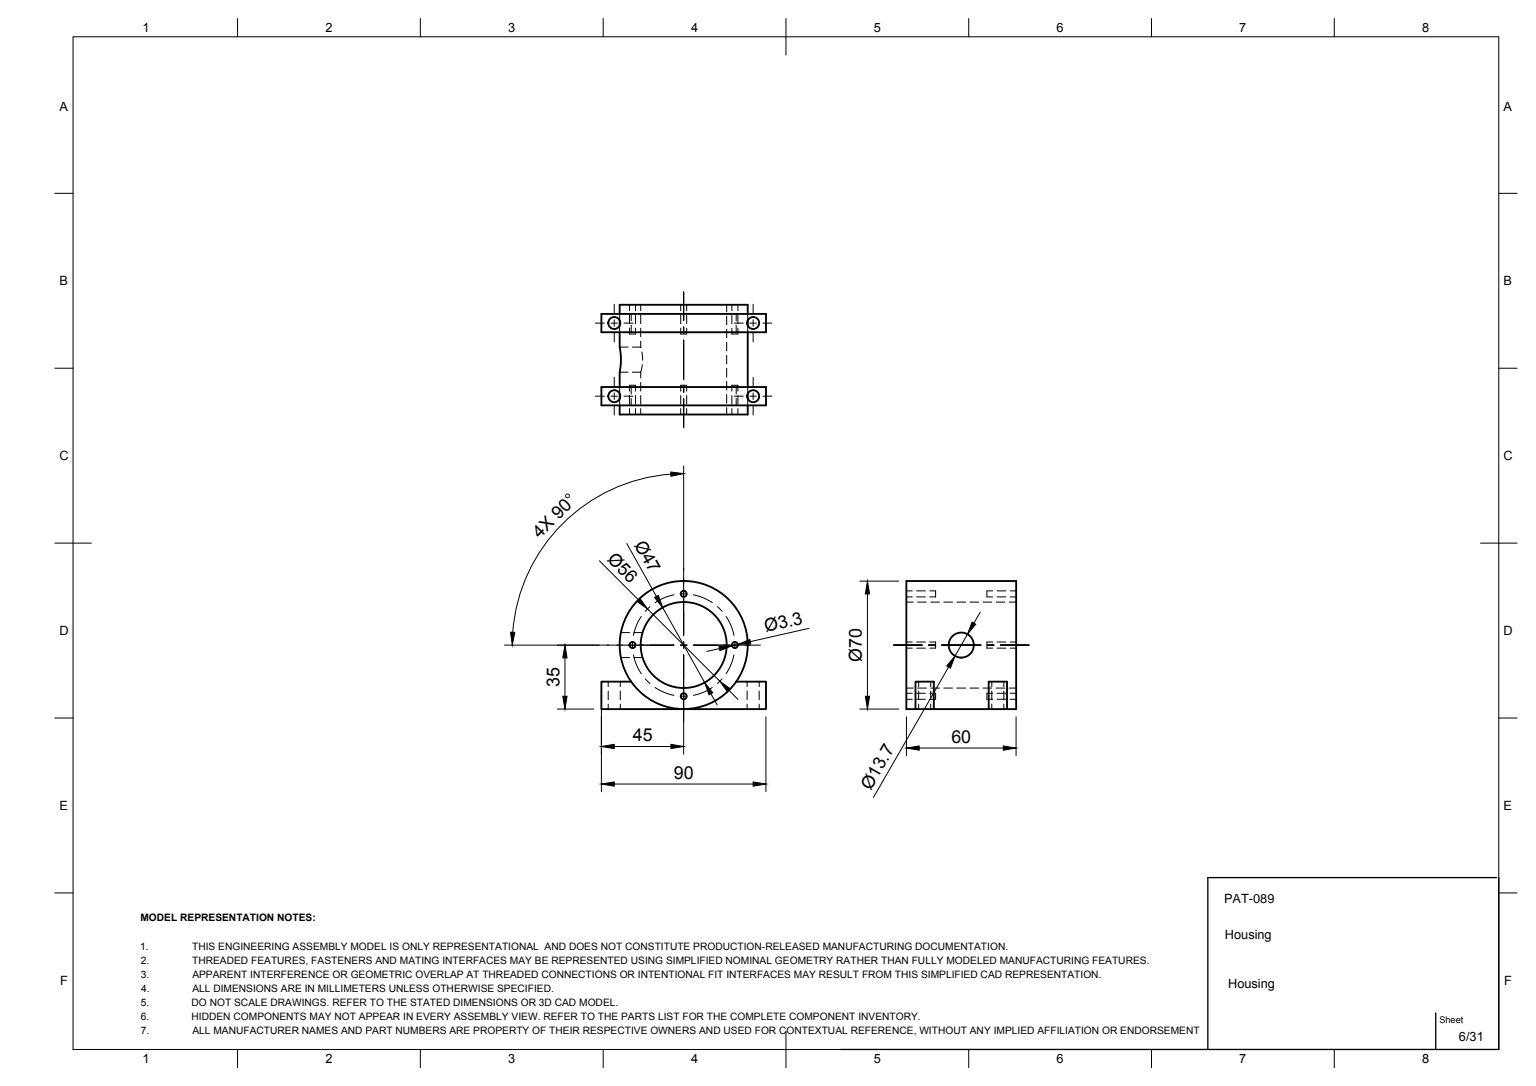
ISO-10303-21;
HEADER;
/* Generated by software containing ST-Developer
 * from STEP Tools, Inc. (www.steptools.com) 
 */

FILE_DESCRIPTION(
/* description */ ('Rotary union on bearing shaft'),
/* implementation_level */ '2;1');

FILE_NAME(
/* name */ 'Housing.step',
/* time_stamp */ '2026-10-28T03:24:01-07:00',
/* author */ (''),
/* organization */ (''),
/* preprocessor_version */ 'ST-DEVELOPER v20.2',
/* originating_system */ 'Autodesk Translation Framework v15.17.0.0',
/* authorisation */ '');

FILE_SCHEMA (('AUTOMOTIVE_DESIGN { 1 0 10303 214 3 1 1 }'));
ENDSEC;

DATA;
#10=MECHANICAL_DESIGN_GEOMETRIC_PRESENTATION_REPRESENTATION('',(#314),#9448);
#225=B_SPLINE_CURVE_WITH_KNOTS('',3,(#7509,#7510,#7511,#7512,#7513,#7514,
#7515,#7516,#7517,#7518,#7519,#7520,#7521,#7522,#7523,#7524,#7525,#7526),
 .UNSPECIFIED.,.F.,.F.,(4,2,2,2,2,2,2,2,4),(0.,0.259699157802782,0.519398315605563,
0.779028864963069,1.03865941432058,1.29828996367808,1.55792051303559,1.81761967083837,
2.07731882864115),.UNSPECIFIED.);
#226=B_SPLINE_CURVE_WITH_KNOTS('',3,(#7527,#7528,#7529,#7530,#7531,#7532,
#7533,#7534,#7535,#7536,#7537,#7538,#7539,#7540,#7541,#7542,#7543,#7544),
 .UNSPECIFIED.,.F.,.F.,(4,2,2,2,2,2,2,2,4),(2.07731882864115,2.33701798644393,
2.59671714424671,2.85634769360422,3.11597824296173,3.37560879231923,3.63523934167674,
3.89493849947952,4.1546376572823),.UNSPECIFIED.);
#227=B_SPLINE_CURVE_WITH_KNOTS('',3,(#7548,#7549,#7550,#7551,#7552,#7553,
#7554,#7555,#7556,#7557,#7558,#7559,#7560,#7561,#7562,#7563,#7564,#7565),
 .UNSPECIFIED.,.F.,.F.,(4,2,2,2,2,2,2,2,4),(0.,0.258756642336745,0.51751328467349,
0.776256652721243,1.035000020769,1.29374338881675,1.5524867568645,1.81124339920125,
2.07000004153799),.UNSPECIFIED.);
#228=B_SPLINE_CURVE_WITH_KNOTS('',3,(#7566,#7567,#7568,#7569,#7570,#7571,
#7572,#7573,#7574,#7575,#7576,#7577,#7578,#7579,#7580,#7581,#7582,#7583),
 .UNSPECIFIED.,.F.,.F.,(4,2,2,2,2,2,2,2,4),(2.07000004153799,2.32875668387474,
2.58751332621148,2.84625669425923,3.10500006230699,3.36374343035474,3.62248679840249,
3.88124344073924,4.14000008307598),.UNSPECIFIED.);
#260=SHAPE_REPRESENTATION_RELATIONSHIP('SRR','None',#9560,#287);
#287=ADVANCED_BREP_SHAPE_REPRESENTATION('',(#349),#9420);
#314=STYLED_ITEM('',(#9757),#349);
#349=MANIFOLD_SOLID_BREP('Body1',#4869);
#388=FACE_BOUND('',#999,.T.);
#389=FACE_BOUND('',#1001,.T.);
#390=FACE_BOUND('',#1004,.T.);
#391=FACE_BOUND('',#1005,.T.);
#392=FACE_BOUND('',#1012,.T.);
#393=FACE_BOUND('',#1014,.T.);
#394=FACE_BOUND('',#1017,.T.);
#395=FACE_BOUND('',#1018,.T.);
#396=FACE_BOUND('',#1021,.T.);
#397=FACE_BOUND('',#1023,.T.);
#398=FACE_BOUND('',#1024,.T.);
#399=FACE_BOUND('',#1025,.T.);
#400=FACE_BOUND('',#1027,.T.);
#401=FACE_BOUND('',#1028,.T.);
#402=FACE_BOUND('',#1029,.T.);
#403=FACE_BOUND('',#1030,.T.);
#404=FACE_BOUND('',#1031,.T.);
#405=FACE_BOUND('',#1033,.T.);
#406=FACE_BOUND('',#1034,.T.);
#407=FACE_BOUND('',#1035,.T.);
#408=FACE_BOUND('',#1036,.T.);
#409=FACE_BOUND('',#1037,.T.);
#493=PLANE('',#5229);
#494=PLANE('',#5233);
#495=PLANE('',#5237);
#496=PLANE('',#5241);
#497=PLANE('',#5245);
#498=PLANE('',#5249);
#499=PLANE('',#5253);
#500=PLANE('',#5257);
#501=PLANE('',#5271);
#502=PLANE('',#5273);
#503=PLANE('',#5275);
#504=PLANE('',#5277);
#505=PLANE('',#5279);
#506=PLANE('',#5280);
#507=PLANE('',#5281);
#508=PLANE('',#5282);
#509=PLANE('',#5283);
#510=PLANE('',#5284);
#511=PLANE('',#5286);
#512=PLANE('',#5288);
#513=PLANE('',#5290);
#514=PLANE('',#5292);
#515=PLANE('',#5293);
#516=PLANE('',#5294);
#517=PLANE('',#5295);
#518=PLANE('',#5296);
#519=PLANE('',#5303);
#520=PLANE('',#5304);
#666=FACE_OUTER_BOUND('',#973,.T.);
#667=FACE_OUTER_BOUND('',#974,.T.);
#668=FACE_OUTER_BOUND('',#975,.T.);
#669=FACE_OUTER_BOUND('',#976,.T.);
#670=FACE_OUTER_BOUND('',#977,.T.);
#671=FACE_OUTER_BOUND('',#978,.T.);
#672=FACE_OUTER_BOUND('',#979,.T.);
#673=FACE_OUTER_BOUND('',#980,.T.);
#674=FACE_OUTER_BOUND('',#981,.T.);
#675=FACE_OUTER_BOUND('',#982,.T.);
#676=FACE_OUTER_BOUND('',#983,.T.);
#677=FACE_OUTER_BOUND('',#984,.T.);
#678=FACE_OUTER_BOUND('',#985,.T.);
#679=FACE_OUTER_BOUND('',#986,.T.);
#680=FACE_OUTER_BOUND('',#987,.T.);
#681=FACE_OUTER_BOUND('',#988,.T.);
#682=FACE_OUTER_BOUND('',#989,.T.);
#683=FACE_OUTER_BOUND('',#990,.T.);
#684=FACE_OUTER_BOUND('',#991,.T.);
#685=FACE_OUTER_BOUND('',#992,.T.);
#686=FACE_OUTER_BOUND('',#993,.T.);
#687=FACE_OUTER_BOUND('',#994,.T.);
#688=FACE_OUTER_BOUND('',#995,.T.);
#689=FACE_OUTER_BOUND('',#996,.T.);
#690=FACE_OUTER_BOUND('',#997,.T.);
#691=FACE_OUTER_BOUND('',#998,.T.);
#692=FACE_OUTER_BOUND('',#1000,.T.);
#693=FACE_OUTER_BOUND('',#1002,.T.);
#694=FACE_OUTER_BOUND('',#1003,.T.);
#695=FACE_OUTER_BOUND('',#1006,.T.);
#696=FACE_OUTER_BOUND('',#1007,.T.);
#697=FACE_OUTER_BOUND('',#1008,.T.);
#698=FACE_OUTER_BOUND('',#1009,.T.);
#699=FACE_OUTER_BOUND('',#1010,.T.);
#700=FACE_OUTER_BOUND('',#1011,.T.);
#701=FACE_OUTER_BOUND('',#1013,.T.);
#702=FACE_OUTER_BOUND('',#1015,.T.);
#703=FACE_OUTER_BOUND('',#1016,.T.);
#704=FACE_OUTER_BOUND('',#1019,.T.);
#705=FACE_OUTER_BOUND('',#1020,.T.);
#706=FACE_OUTER_BOUND('',#1022,.T.);
#707=FACE_OUTER_BOUND('',#1026,.T.);
#708=FACE_OUTER_BOUND('',#1032,.T.);
#973=EDGE_LOOP('',(#3315,#3316,#3317,#3318));
#974=EDGE_LOOP('',(#3319));
#975=EDGE_LOOP('',(#3320,#3321,#3322,#3323));
#976=EDGE_LOOP('',(#3324));
#977=EDGE_LOOP('',(#3325,#3326,#3327,#3328));
#978=EDGE_LOOP('',(#3329));
#979=EDGE_LOOP('',(#3330,#3331,#3332,#3333));
#980=EDGE_LOOP('',(#3334));
#981=EDGE_LOOP('',(#3335,#3336,#3337,#3338));
#982=EDGE_LOOP('',(#3339));
#983=EDGE_LOOP('',(#3340,#3341,#3342,#3343));
#984=EDGE_LOOP('',(#3344));
#985=EDGE_LOOP('',(#3345,#3346,#3347,#3348));
#986=EDGE_LOOP('',(#3349));
#987=EDGE_LOOP('',(#3350,#3351,#3352,#3353));
#988=EDGE_LOOP('',(#3354));
#989=EDGE_LOOP('',(#3355,#3356,#3357,#3358,#3359,#3360));
#990=EDGE_LOOP('',(#3361,#3362,#3363,#3364));
#991=EDGE_LOOP('',(#3365,#3366,#3367,#3368));
#992=EDGE_LOOP('',(#3369,#3370,#3371,#3372));
#993=EDGE_LOOP('',(#3373,#3374,#3375,#3376));
#994=EDGE_LOOP('',(#3377,#3378,#3379,#3380));
#995=EDGE_LOOP('',(#3381,#3382,#3383,#3384));
#996=EDGE_LOOP('',(#3385,#3386,#3387,#3388));
#997=EDGE_LOOP('',(#3389,#3390,#3391,#3392));
#998=EDGE_LOOP('',(#3393,#3394,#3395,#3396));
#999=EDGE_LOOP('',(#3397));
#1000=EDGE_LOOP('',(#3398,#3399,#3400,#3401));
#1001=EDGE_LOOP('',(#3402));
#1002=EDGE_LOOP('',(#3403,#3404,#3405,#3406));
#1003=EDGE_LOOP('',(#3407,#3408,#3409,#3410,#3411,#3412));
#1004=EDGE_LOOP('',(#3413));
#1005=EDGE_LOOP('',(#3414));
#1006=EDGE_LOOP('',(#3415,#3416,#3417,#3418));
#1007=EDGE_LOOP('',(#3419,#3420,#3421,#3422));
#1008=EDGE_LOOP('',(#3423,#3424,#3425,#3426));
#1009=EDGE_LOOP('',(#3427,#3428,#3429,#3430));
#1010=EDGE_LOOP('',(#3431,#3432,#3433,#3434));
#1011=EDGE_LOOP('',(#3435,#3436,#3437,#3438));
#1012=EDGE_LOOP('',(#3439));
#1013=EDGE_LOOP('',(#3440,#3441,#3442,#3443));
#1014=EDGE_LOOP('',(#3444));
#1015=EDGE_LOOP('',(#3445,#3446,#3447,#3448));
#1016=EDGE_LOOP('',(#3449,#3450,#3451,#3452,#3453,#3454));
#1017=EDGE_LOOP('',(#3455));
#1018=EDGE_LOOP('',(#3456));
#1019=EDGE_LOOP('',(#3457,#3458,#3459,#3460));
#1020=EDGE_LOOP('',(#3461,#3462,#3463,#3464));
#1021=EDGE_LOOP('',(#3465,#3466));
#1022=EDGE_LOOP('',(#3467,#3468,#3469,#3470));
#1023=EDGE_LOOP('',(#3471,#3472));
#1024=EDGE_LOOP('',(#3473,#3474,#3475,#3476,#3477,#3478));
#1025=EDGE_LOOP('',(#3479,#3480,#3481,#3482,#3483,#3484));
#1026=EDGE_LOOP('',(#3485));
#1027=EDGE_LOOP('',(#3486));
#1028=EDGE_LOOP('',(#3487));
#1029=EDGE_LOOP('',(#3488));
#1030=EDGE_LOOP('',(#3489));
#1031=EDGE_LOOP('',(#3490));
#1032=EDGE_LOOP('',(#3491));
#1033=EDGE_LOOP('',(#3492));
#1034=EDGE_LOOP('',(#3493));
#1035=EDGE_LOOP('',(#3494));
#1036=EDGE_LOOP('',(#3495));
#1037=EDGE_LOOP('',(#3496));
#1377=LINE('',#7454,#1697);
#1378=LINE('',#7461,#1698);
#1379=LINE('',#7468,#1699);
#1380=LINE('',#7475,#1700);
#1381=LINE('',#7482,#1701);
#1382=LINE('',#7489,#1702);
#1383=LINE('',#7496,#1703);
#1384=LINE('',#7503,#1704);
#1385=LINE('',#7546,#1705);
#1386=LINE('',#7588,#1706);
#1387=LINE('',#7594,#1707);
#1388=LINE('',#7600,#1708);
#1389=LINE('',#7606,#1709);
#1390=LINE('',#7613,#1710);
#1391=LINE('',#7615,#1711);
#1392=LINE('',#7616,#1712);
#1393=LINE('',#7621,#1713);
#1394=LINE('',#7623,#1714);
#1395=LINE('',#7624,#1715);
#1396=LINE('',#7630,#1716);
#1397=LINE('',#7632,#1717);
#1398=LINE('',#7633,#1718);
#1399=LINE('',#7638,#1719);
#1400=LINE('',#7640,#1720);
#1401=LINE('',#7641,#1721);
#1402=LINE('',#7643,#1722);
#1403=LINE('',#7644,#1723);
#1404=LINE('',#7646,#1724);
#1405=LINE('',#7647,#1725);
#1406=LINE('',#7649,#1726);
#1407=LINE('',#7651,#1727);
#1408=LINE('',#7658,#1728);
#1409=LINE('',#7660,#1729);
#1410=LINE('',#7661,#1730);
#1411=LINE('',#7666,#1731);
#1412=LINE('',#7668,#1732);
#1413=LINE('',#7669,#1733);
#1414=LINE('',#7675,#1734);
#1415=LINE('',#7677,#1735);
#1416=LINE('',#7678,#1736);
#1417=LINE('',#7683,#1737);
#1418=LINE('',#7685,#1738);
#1419=LINE('',#7686,#1739);
#1420=LINE('',#7688,#1740);
#1421=LINE('',#7689,#1741);
#1422=LINE('',#7691,#1742);
#1423=LINE('',#7692,#1743);
#1424=LINE('',#7694,#1744);
#1425=LINE('',#7696,#1745);
#1426=LINE('',#7702,#1746);
#1427=LINE('',#7708,#1747);
#1697=VECTOR('',#5892,0.165);
#1698=VECTOR('',#5901,0.165);
#1699=VECTOR('',#5910,0.165);
#1700=VECTOR('',#5919,0.165);
#1701=VECTOR('',#5928,0.165);
#1702=VECTOR('',#5937,0.165);
#1703=VECTOR('',#5946,0.165);
#1704=VECTOR('',#5955,0.165);
#1705=VECTOR('',#5962,0.685);
#1706=VECTOR('',#5967,0.33);
#1707=VECTOR('',#5974,0.33);
#1708=VECTOR('',#5981,0.33);
#1709=VECTOR('',#5988,0.33);
#1710=VECTOR('',#5995,1.);
#1711=VECTOR('',#5996,1.);
#1712=VECTOR('',#5997,1.);
#1713=VECTOR('',#6002,1.);
#1714=VECTOR('',#6003,1.);
#1715=VECTOR('',#6004,1.);
#1716=VECTOR('',#6009,1.);
#1717=VECTOR('',#6010,1.);
#1718=VECTOR('',#6011,1.);
#1719=VECTOR('',#6016,1.);
#1720=VECTOR('',#6017,1.);
#1721=VECTOR('',#6018,1.);
#1722=VECTOR('',#6021,1.);
#1723=VECTOR('',#6022,1.);
#1724=VECTOR('',#6025,1.);
#1725=VECTOR('',#6026,1.);
#1726=VECTOR('',#6029,1.);
#1727=VECTOR('',#6032,1.);
#1728=VECTOR('',#6039,1.);
#1729=VECTOR('',#6040,1.);
#1730=VECTOR('',#6041,1.);
#1731=VECTOR('',#6046,1.);
#1732=VECTOR('',#6047,1.);
#1733=VECTOR('',#6048,1.);
#1734=VECTOR('',#6053,1.);
#1735=VECTOR('',#6054,1.);
#1736=VECTOR('',#6055,1.);
#1737=VECTOR('',#6060,1.);
#1738=VECTOR('',#6061,1.);
#1739=VECTOR('',#6062,1.);
#1740=VECTOR('',#6065,1.);
#1741=VECTOR('',#6066,1.);
#1742=VECTOR('',#6069,1.);
#1743=VECTOR('',#6070,1.);
#1744=VECTOR('',#6073,1.);
#1745=VECTOR('',#6076,1.);
#1746=VECTOR('',#6083,2.35);
#1747=VECTOR('',#6090,3.5);
#2009=CIRCLE('',#5227,0.165);
#2010=CIRCLE('',#5228,0.165);
#2011=CIRCLE('',#5231,0.165);
#2012=CIRCLE('',#5232,0.165);
#2013=CIRCLE('',#5235,0.165);
#2014=CIRCLE('',#5236,0.165);
#2015=CIRCLE('',#5239,0.165);
#2016=CIRCLE('',#5240,0.165);
#2017=CIRCLE('',#5243,0.165);
#2018=CIRCLE('',#5244,0.165);
#2019=CIRCLE('',#5247,0.165);
#2020=CIRCLE('',#5248,0.165);
#2021=CIRCLE('',#5251,0.165);
#2022=CIRCLE('',#5252,0.165);
#2023=CIRCLE('',#5255,0.165);
#2024=CIRCLE('',#5256,0.165);
#2025=CIRCLE('',#5260,0.33);
#2026=CIRCLE('',#5261,0.33);
#2027=CIRCLE('',#5263,0.33);
#2028=CIRCLE('',#5264,0.33);
#2029=CIRCLE('',#5266,0.33);
#2030=CIRCLE('',#5267,0.33);
#2031=CIRCLE('',#5269,0.33);
#2032=CIRCLE('',#5270,0.33);
#2033=CIRCLE('',#5272,3.5);
#2034=CIRCLE('',#5274,3.5);
#2035=CIRCLE('',#5276,3.5);
#2036=CIRCLE('',#5278,3.5);
#2037=CIRCLE('',#5285,3.5);
#2038=CIRCLE('',#5287,3.5);
#2039=CIRCLE('',#5289,3.5);
#2040=CIRCLE('',#5291,3.5);
#2041=CIRCLE('',#5298,2.35);
#2042=CIRCLE('',#5299,2.35);
#2043=CIRCLE('',#5301,3.5);
#2044=CIRCLE('',#5302,3.5);
#2269=VERTEX_POINT('',#7451);
#2270=VERTEX_POINT('',#7453);
#2271=VERTEX_POINT('',#7458);
#2272=VERTEX_POINT('',#7460);
#2273=VERTEX_POINT('',#7465);
#2274=VERTEX_POINT('',#7467);
#2275=VERTEX_POINT('',#7472);
#2276=VERTEX_POINT('',#7474);
#2277=VERTEX_POINT('',#7479);
#2278=VERTEX_POINT('',#7481);
#2279=VERTEX_POINT('',#7486);
#2280=VERTEX_POINT('',#7488);
#2281=VERTEX_POINT('',#7493);
#2282=VERTEX_POINT('',#7495);
#2283=VERTEX_POINT('',#7500);
#2284=VERTEX_POINT('',#7502);
#2285=VERTEX_POINT('',#7507);
#2286=VERTEX_POINT('',#7508);
#2287=VERTEX_POINT('',#7545);
#2288=VERTEX_POINT('',#7547);
#2289=VERTEX_POINT('',#7585);
#2290=VERTEX_POINT('',#7587);
#2291=VERTEX_POINT('',#7591);
#2292=VERTEX_POINT('',#7593);
#2293=VERTEX_POINT('',#7597);
#2294=VERTEX_POINT('',#7599);
#2295=VERTEX_POINT('',#7603);
#2296=VERTEX_POINT('',#7605);
#2297=VERTEX_POINT('',#7609);
#2298=VERTEX_POINT('',#7610);
#2299=VERTEX_POINT('',#7612);
#2300=VERTEX_POINT('',#7614);
#2301=VERTEX_POINT('',#7618);
#2302=VERTEX_POINT('',#7620);
#2303=VERTEX_POINT('',#7622);
#2304=VERTEX_POINT('',#7626);
#2305=VERTEX_POINT('',#7627);
#2306=VERTEX_POINT('',#7629);
#2307=VERTEX_POINT('',#7631);
#2308=VERTEX_POINT('',#7635);
#2309=VERTEX_POINT('',#7637);
#2310=VERTEX_POINT('',#7639);
#2311=VERTEX_POINT('',#7654);
#2312=VERTEX_POINT('',#7655);
#2313=VERTEX_POINT('',#7657);
#2314=VERTEX_POINT('',#7659);
#2315=VERTEX_POINT('',#7663);
#2316=VERTEX_POINT('',#7665);
#2317=VERTEX_POINT('',#7667);
#2318=VERTEX_POINT('',#7671);
#2319=VERTEX_POINT('',#7672);
#2320=VERTEX_POINT('',#7674);
#2321=VERTEX_POINT('',#7676);
#2322=VERTEX_POINT('',#7680);
#2323=VERTEX_POINT('',#7682);
#2324=VERTEX_POINT('',#7684);
#2325=VERTEX_POINT('',#7699);
#2326=VERTEX_POINT('',#7701);
#2327=VERTEX_POINT('',#7705);
#2328=VERTEX_POINT('',#7707);
#2685=EDGE_CURVE('',#2269,#2269,#2009,.T.);
#2686=EDGE_CURVE('',#2269,#2270,#1377,.T.);
#2687=EDGE_CURVE('',#2270,#2270,#2010,.T.);
#2688=EDGE_CURVE('',#2271,#2271,#2011,.T.);
#2689=EDGE_CURVE('',#2271,#2272,#1378,.T.);
#2690=EDGE_CURVE('',#2272,#2272,#2012,.T.);
#2691=EDGE_CURVE('',#2273,#2273,#2013,.T.);
#2692=EDGE_CURVE('',#2273,#2274,#1379,.T.);
#2693=EDGE_CURVE('',#2274,#2274,#2014,.T.);
#2694=EDGE_CURVE('',#2275,#2275,#2015,.T.);
#2695=EDGE_CURVE('',#2275,#2276,#1380,.T.);
#2696=EDGE_CURVE('',#2276,#2276,#2016,.T.);
#2697=EDGE_CURVE('',#2277,#2277,#2017,.T.);
#2698=EDGE_CURVE('',#2277,#2278,#1381,.T.);
#2699=EDGE_CURVE('',#2278,#2278,#2018,.T.);
#2700=EDGE_CURVE('',#2279,#2279,#2019,.T.);
#2701=EDGE_CURVE('',#2279,#2280,#1382,.T.);
#2702=EDGE_CURVE('',#2280,#2280,#2020,.T.);
#2703=EDGE_CURVE('',#2281,#2281,#2021,.T.);
#2704=EDGE_CURVE('',#2281,#2282,#1383,.T.);
#2705=EDGE_CURVE('',#2282,#2282,#2022,.T.);
#2706=EDGE_CURVE('',#2283,#2283,#2023,.T.);
#2707=EDGE_CURVE('',#2283,#2284,#1384,.T.);
#2708=EDGE_CURVE('',#2284,#2284,#2024,.T.);
#2709=EDGE_CURVE('',#2285,#2286,#225,.T.);
#2710=EDGE_CURVE('',#2286,#2285,#226,.T.);
#2711=EDGE_CURVE('',#2286,#2287,#1385,.T.);
#2712=EDGE_CURVE('',#2288,#2287,#227,.T.);
#2713=EDGE_CURVE('',#2287,#2288,#228,.T.);
#2714=EDGE_CURVE('',#2289,#2289,#2025,.T.);
#2715=EDGE_CURVE('',#2289,#2290,#1386,.T.);
#2716=EDGE_CURVE('',#2290,#2290,#2026,.T.);
#2717=EDGE_CURVE('',#2291,#2291,#2027,.T.);
#2718=EDGE_CURVE('',#2291,#2292,#1387,.T.);
#2719=EDGE_CURVE('',#2292,#2292,#2028,.T.);
#2720=EDGE_CURVE('',#2293,#2293,#2029,.T.);
#2721=EDGE_CURVE('',#2293,#2294,#1388,.T.);
#2722=EDGE_CURVE('',#2294,#2294,#2030,.T.);
#2723=EDGE_CURVE('',#2295,#2295,#2031,.T.);
#2724=EDGE_CURVE('',#2295,#2296,#1389,.T.);
#2725=EDGE_CURVE('',#2296,#2296,#2032,.T.);
#2726=EDGE_CURVE('',#2297,#2298,#2033,.T.);
#2727=EDGE_CURVE('',#2297,#2299,#1390,.T.);
#2728=EDGE_CURVE('',#2299,#2300,#1391,.T.);
#2729=EDGE_CURVE('',#2300,#2298,#1392,.T.);
#2730=EDGE_CURVE('',#2298,#2301,#2034,.T.);
#2731=EDGE_CURVE('',#2298,#2302,#1393,.T.);
#2732=EDGE_CURVE('',#2302,#2303,#1394,.T.);
#2733=EDGE_CURVE('',#2303,#2301,#1395,.T.);
#2734=EDGE_CURVE('',#2304,#2305,#2035,.T.);
#2735=EDGE_CURVE('',#2304,#2306,#1396,.T.);
#2736=EDGE_CURVE('',#2306,#2307,#1397,.T.);
#2737=EDGE_CURVE('',#2307,#2305,#1398,.T.);
#2738=EDGE_CURVE('',#2308,#2304,#2036,.T.);
#2739=EDGE_CURVE('',#2308,#2309,#1399,.T.);
#2740=EDGE_CURVE('',#2309,#2310,#1400,.T.);
#2741=EDGE_CURVE('',#2310,#2304,#1401,.T.);
#2742=EDGE_CURVE('',#2305,#2297,#1402,.T.);
#2743=EDGE_CURVE('',#2307,#2299,#1403,.T.);
#2744=EDGE_CURVE('',#2301,#2308,#1404,.T.);
#2745=EDGE_CURVE('',#2309,#2303,#1405,.T.);
#2746=EDGE_CURVE('',#2310,#2302,#1406,.T.);
#2747=EDGE_CURVE('',#2306,#2300,#1407,.T.);
#2748=EDGE_CURVE('',#2311,#2312,#2037,.T.);
#2749=EDGE_CURVE('',#2311,#2313,#1408,.T.);
#2750=EDGE_CURVE('',#2313,#2314,#1409,.T.);
#2751=EDGE_CURVE('',#2314,#2312,#1410,.T.);
#2752=EDGE_CURVE('',#2312,#2315,#2038,.T.);
#2753=EDGE_CURVE('',#2312,#2316,#1411,.T.);
#2754=EDGE_CURVE('',#2316,#2317,#1412,.T.);
#2755=EDGE_CURVE('',#2317,#2315,#1413,.T.);
#2756=EDGE_CURVE('',#2318,#2319,#2039,.T.);
#2757=EDGE_CURVE('',#2318,#2320,#1414,.T.);
#2758=EDGE_CURVE('',#2320,#2321,#1415,.T.);
#2759=EDGE_CURVE('',#2321,#2319,#1416,.T.);
#2760=EDGE_CURVE('',#2322,#2318,#2040,.T.);
#2761=EDGE_CURVE('',#2322,#2323,#1417,.T.);
#2762=EDGE_CURVE('',#2323,#2324,#1418,.T.);
#2763=EDGE_CURVE('',#2324,#2318,#1419,.T.);
#2764=EDGE_CURVE('',#2319,#2311,#1420,.T.);
#2765=EDGE_CURVE('',#2321,#2313,#1421,.T.);
#2766=EDGE_CURVE('',#2315,#2322,#1422,.T.);
#2767=EDGE_CURVE('',#2323,#2317,#1423,.T.);
#2768=EDGE_CURVE('',#2324,#2316,#1424,.T.);
#2769=EDGE_CURVE('',#2320,#2314,#1425,.T.);
#2770=EDGE_CURVE('',#2325,#2325,#2041,.T.);
#2771=EDGE_CURVE('',#2325,#2326,#1426,.T.);
#2772=EDGE_CURVE('',#2326,#2326,#2042,.T.);
#2773=EDGE_CURVE('',#2327,#2327,#2043,.T.);
#2774=EDGE_CURVE('',#2327,#2328,#1427,.T.);
#2775=EDGE_CURVE('',#2328,#2328,#2044,.T.);
#3315=ORIENTED_EDGE('',*,*,#2685,.F.);
#3316=ORIENTED_EDGE('',*,*,#2686,.T.);
#3317=ORIENTED_EDGE('',*,*,#2687,.F.);
#3318=ORIENTED_EDGE('',*,*,#2686,.F.);
#3319=ORIENTED_EDGE('',*,*,#2685,.T.);
#3320=ORIENTED_EDGE('',*,*,#2688,.F.);
#3321=ORIENTED_EDGE('',*,*,#2689,.T.);
#3322=ORIENTED_EDGE('',*,*,#2690,.F.);
#3323=ORIENTED_EDGE('',*,*,#2689,.F.);
#3324=ORIENTED_EDGE('',*,*,#2688,.T.);
#3325=ORIENTED_EDGE('',*,*,#2691,.F.);
#3326=ORIENTED_EDGE('',*,*,#2692,.T.);
#3327=ORIENTED_EDGE('',*,*,#2693,.F.);
#3328=ORIENTED_EDGE('',*,*,#2692,.F.);
#3329=ORIENTED_EDGE('',*,*,#2691,.T.);
#3330=ORIENTED_EDGE('',*,*,#2694,.F.);
#3331=ORIENTED_EDGE('',*,*,#2695,.T.);
#3332=ORIENTED_EDGE('',*,*,#2696,.F.);
#3333=ORIENTED_EDGE('',*,*,#2695,.F.);
#3334=ORIENTED_EDGE('',*,*,#2694,.T.);
#3335=ORIENTED_EDGE('',*,*,#2697,.F.);
#3336=ORIENTED_EDGE('',*,*,#2698,.T.);
#3337=ORIENTED_EDGE('',*,*,#2699,.T.);
#3338=ORIENTED_EDGE('',*,*,#2698,.F.);
#3339=ORIENTED_EDGE('',*,*,#2699,.F.);
#3340=ORIENTED_EDGE('',*,*,#2700,.F.);
#3341=ORIENTED_EDGE('',*,*,#2701,.T.);
#3342=ORIENTED_EDGE('',*,*,#2702,.T.);
#3343=ORIENTED_EDGE('',*,*,#2701,.F.);
#3344=ORIENTED_EDGE('',*,*,#2702,.F.);
#3345=ORIENTED_EDGE('',*,*,#2703,.F.);
#3346=ORIENTED_EDGE('',*,*,#2704,.T.);
#3347=ORIENTED_EDGE('',*,*,#2705,.T.);
#3348=ORIENTED_EDGE('',*,*,#2704,.F.);
#3349=ORIENTED_EDGE('',*,*,#2705,.F.);
#3350=ORIENTED_EDGE('',*,*,#2706,.F.);
#3351=ORIENTED_EDGE('',*,*,#2707,.T.);
#3352=ORIENTED_EDGE('',*,*,#2708,.T.);
#3353=ORIENTED_EDGE('',*,*,#2707,.F.);
#3354=ORIENTED_EDGE('',*,*,#2708,.F.);
#3355=ORIENTED_EDGE('',*,*,#2709,.F.);
#3356=ORIENTED_EDGE('',*,*,#2710,.F.);
#3357=ORIENTED_EDGE('',*,*,#2711,.T.);
#3358=ORIENTED_EDGE('',*,*,#2712,.F.);
#3359=ORIENTED_EDGE('',*,*,#2713,.F.);
#3360=ORIENTED_EDGE('',*,*,#2711,.F.);
#3361=ORIENTED_EDGE('',*,*,#2714,.F.);
#3362=ORIENTED_EDGE('',*,*,#2715,.T.);
#3363=ORIENTED_EDGE('',*,*,#2716,.F.);
#3364=ORIENTED_EDGE('',*,*,#2715,.F.);
#3365=ORIENTED_EDGE('',*,*,#2717,.F.);
#3366=ORIENTED_EDGE('',*,*,#2718,.T.);
#3367=ORIENTED_EDGE('',*,*,#2719,.F.);
#3368=ORIENTED_EDGE('',*,*,#2718,.F.);
#3369=ORIENTED_EDGE('',*,*,#2720,.F.);
#3370=ORIENTED_EDGE('',*,*,#2721,.T.);
#3371=ORIENTED_EDGE('',*,*,#2722,.F.);
#3372=ORIENTED_EDGE('',*,*,#2721,.F.);
#3373=ORIENTED_EDGE('',*,*,#2723,.F.);
#3374=ORIENTED_EDGE('',*,*,#2724,.T.);
#3375=ORIENTED_EDGE('',*,*,#2725,.F.);
#3376=ORIENTED_EDGE('',*,*,#2724,.F.);
#3377=ORIENTED_EDGE('',*,*,#2726,.F.);
#3378=ORIENTED_EDGE('',*,*,#2727,.T.);
#3379=ORIENTED_EDGE('',*,*,#2728,.T.);
#3380=ORIENTED_EDGE('',*,*,#2729,.T.);
#3381=ORIENTED_EDGE('',*,*,#2730,.F.);
#3382=ORIENTED_EDGE('',*,*,#2731,.T.);
#3383=ORIENTED_EDGE('',*,*,#2732,.T.);
#3384=ORIENTED_EDGE('',*,*,#2733,.T.);
#3385=ORIENTED_EDGE('',*,*,#2734,.F.);
#3386=ORIENTED_EDGE('',*,*,#2735,.T.);
#3387=ORIENTED_EDGE('',*,*,#2736,.T.);
#3388=ORIENTED_EDGE('',*,*,#2737,.T.);
#3389=ORIENTED_EDGE('',*,*,#2738,.F.);
#3390=ORIENTED_EDGE('',*,*,#2739,.T.);
#3391=ORIENTED_EDGE('',*,*,#2740,.T.);
#3392=ORIENTED_EDGE('',*,*,#2741,.T.);
#3393=ORIENTED_EDGE('',*,*,#2742,.F.);
#3394=ORIENTED_EDGE('',*,*,#2737,.F.);
#3395=ORIENTED_EDGE('',*,*,#2743,.T.);
#3396=ORIENTED_EDGE('',*,*,#2727,.F.);
#3397=ORIENTED_EDGE('',*,*,#2725,.T.);
#3398=ORIENTED_EDGE('',*,*,#2744,.F.);
#3399=ORIENTED_EDGE('',*,*,#2733,.F.);
#3400=ORIENTED_EDGE('',*,*,#2745,.F.);
#3401=ORIENTED_EDGE('',*,*,#2739,.F.);
#3402=ORIENTED_EDGE('',*,*,#2719,.T.);
#3403=ORIENTED_EDGE('',*,*,#2740,.F.);
#3404=ORIENTED_EDGE('',*,*,#2745,.T.);
#3405=ORIENTED_EDGE('',*,*,#2732,.F.);
#3406=ORIENTED_EDGE('',*,*,#2746,.F.);
#3407=ORIENTED_EDGE('',*,*,#2729,.F.);
#3408=ORIENTED_EDGE('',*,*,#2747,.F.);
#3409=ORIENTED_EDGE('',*,*,#2735,.F.);
#3410=ORIENTED_EDGE('',*,*,#2741,.F.);
#3411=ORIENTED_EDGE('',*,*,#2746,.T.);
#3412=ORIENTED_EDGE('',*,*,#2731,.F.);
#3413=ORIENTED_EDGE('',*,*,#2717,.T.);
#3414=ORIENTED_EDGE('',*,*,#2723,.T.);
#3415=ORIENTED_EDGE('',*,*,#2736,.F.);
#3416=ORIENTED_EDGE('',*,*,#2747,.T.);
#3417=ORIENTED_EDGE('',*,*,#2728,.F.);
#3418=ORIENTED_EDGE('',*,*,#2743,.F.);
#3419=ORIENTED_EDGE('',*,*,#2748,.F.);
#3420=ORIENTED_EDGE('',*,*,#2749,.T.);
#3421=ORIENTED_EDGE('',*,*,#2750,.T.);
#3422=ORIENTED_EDGE('',*,*,#2751,.T.);
#3423=ORIENTED_EDGE('',*,*,#2752,.F.);
#3424=ORIENTED_EDGE('',*,*,#2753,.T.);
#3425=ORIENTED_EDGE('',*,*,#2754,.T.);
#3426=ORIENTED_EDGE('',*,*,#2755,.T.);
#3427=ORIENTED_EDGE('',*,*,#2756,.F.);
#3428=ORIENTED_EDGE('',*,*,#2757,.T.);
#3429=ORIENTED_EDGE('',*,*,#2758,.T.);
#3430=ORIENTED_EDGE('',*,*,#2759,.T.);
#3431=ORIENTED_EDGE('',*,*,#2760,.F.);
#3432=ORIENTED_EDGE('',*,*,#2761,.T.);
#3433=ORIENTED_EDGE('',*,*,#2762,.T.);
#3434=ORIENTED_EDGE('',*,*,#2763,.T.);
#3435=ORIENTED_EDGE('',*,*,#2764,.F.);
#3436=ORIENTED_EDGE('',*,*,#2759,.F.);
#3437=ORIENTED_EDGE('',*,*,#2765,.T.);
#3438=ORIENTED_EDGE('',*,*,#2749,.F.);
#3439=ORIENTED_EDGE('',*,*,#2716,.T.);
#3440=ORIENTED_EDGE('',*,*,#2766,.F.);
#3441=ORIENTED_EDGE('',*,*,#2755,.F.);
#3442=ORIENTED_EDGE('',*,*,#2767,.F.);
#3443=ORIENTED_EDGE('',*,*,#2761,.F.);
#3444=ORIENTED_EDGE('',*,*,#2722,.T.);
#3445=ORIENTED_EDGE('',*,*,#2762,.F.);
#3446=ORIENTED_EDGE('',*,*,#2767,.T.);
#3447=ORIENTED_EDGE('',*,*,#2754,.F.);
#3448=ORIENTED_EDGE('',*,*,#2768,.F.);
#3449=ORIENTED_EDGE('',*,*,#2751,.F.);
#3450=ORIENTED_EDGE('',*,*,#2769,.F.);
#3451=ORIENTED_EDGE('',*,*,#2757,.F.);
#3452=ORIENTED_EDGE('',*,*,#2763,.F.);
#3453=ORIENTED_EDGE('',*,*,#2768,.T.);
#3454=ORIENTED_EDGE('',*,*,#2753,.F.);
#3455=ORIENTED_EDGE('',*,*,#2714,.T.);
#3456=ORIENTED_EDGE('',*,*,#2720,.T.);
#3457=ORIENTED_EDGE('',*,*,#2758,.F.);
#3458=ORIENTED_EDGE('',*,*,#2769,.T.);
#3459=ORIENTED_EDGE('',*,*,#2750,.F.);
#3460=ORIENTED_EDGE('',*,*,#2765,.F.);
#3461=ORIENTED_EDGE('',*,*,#2770,.F.);
#3462=ORIENTED_EDGE('',*,*,#2771,.T.);
#3463=ORIENTED_EDGE('',*,*,#2772,.T.);
#3464=ORIENTED_EDGE('',*,*,#2771,.F.);
#3465=ORIENTED_EDGE('',*,*,#2709,.T.);
#3466=ORIENTED_EDGE('',*,*,#2710,.T.);
#3467=ORIENTED_EDGE('',*,*,#2773,.F.);
#3468=ORIENTED_EDGE('',*,*,#2774,.T.);
#3469=ORIENTED_EDGE('',*,*,#2775,.T.);
#3470=ORIENTED_EDGE('',*,*,#2774,.F.);
#3471=ORIENTED_EDGE('',*,*,#2712,.T.);
#3472=ORIENTED_EDGE('',*,*,#2713,.T.);
#3473=ORIENTED_EDGE('',*,*,#2742,.T.);
#3474=ORIENTED_EDGE('',*,*,#2726,.T.);
#3475=ORIENTED_EDGE('',*,*,#2730,.T.);
#3476=ORIENTED_EDGE('',*,*,#2744,.T.);
#3477=ORIENTED_EDGE('',*,*,#2738,.T.);
#3478=ORIENTED_EDGE('',*,*,#2734,.T.);
#3479=ORIENTED_EDGE('',*,*,#2764,.T.);
#3480=ORIENTED_EDGE('',*,*,#2748,.T.);
#3481=ORIENTED_EDGE('',*,*,#2752,.T.);
#3482=ORIENTED_EDGE('',*,*,#2766,.T.);
#3483=ORIENTED_EDGE('',*,*,#2760,.T.);
#3484=ORIENTED_EDGE('',*,*,#2756,.T.);
#3485=ORIENTED_EDGE('',*,*,#2773,.T.);
#3486=ORIENTED_EDGE('',*,*,#2770,.T.);
#3487=ORIENTED_EDGE('',*,*,#2696,.T.);
#3488=ORIENTED_EDGE('',*,*,#2693,.T.);
#3489=ORIENTED_EDGE('',*,*,#2690,.T.);
#3490=ORIENTED_EDGE('',*,*,#2687,.T.);
#3491=ORIENTED_EDGE('',*,*,#2775,.F.);
#3492=ORIENTED_EDGE('',*,*,#2772,.F.);
#3493=ORIENTED_EDGE('',*,*,#2706,.T.);
#3494=ORIENTED_EDGE('',*,*,#2703,.T.);
#3495=ORIENTED_EDGE('',*,*,#2700,.T.);
#3496=ORIENTED_EDGE('',*,*,#2697,.T.);
#4483=CYLINDRICAL_SURFACE('',#5226,0.165);
#4484=CYLINDRICAL_SURFACE('',#5230,0.165);
#4485=CYLINDRICAL_SURFACE('',#5234,0.165);
#4486=CYLINDRICAL_SURFACE('',#5238,0.165);
#4487=CYLINDRICAL_SURFACE('',#5242,0.165);
#4488=CYLINDRICAL_SURFACE('',#5246,0.165);
#4489=CYLINDRICAL_SURFACE('',#5250,0.165);
#4490=CYLINDRICAL_SURFACE('',#5254,0.165);
#4491=CYLINDRICAL_SURFACE('',#5258,0.685);
#4492=CYLINDRICAL_SURFACE('',#5259,0.33);
#4493=CYLINDRICAL_SURFACE('',#5262,0.33);
#4494=CYLINDRICAL_SURFACE('',#5265,0.33);
#4495=CYLINDRICAL_SURFACE('',#5268,0.33);
#4496=CYLINDRICAL_SURFACE('',#5297,2.35);
#4497=CYLINDRICAL_SURFACE('',#5300,3.5);
#4579=ADVANCED_FACE('',(#666),#4483,.F.);
#4580=ADVANCED_FACE('',(#667),#493,.T.);
#4581=ADVANCED_FACE('',(#668),#4484,.F.);
#4582=ADVANCED_FACE('',(#669),#494,.T.);
#4583=ADVANCED_FACE('',(#670),#4485,.F.);
#4584=ADVANCED_FACE('',(#671),#495,.T.);
#4585=ADVANCED_FACE('',(#672),#4486,.F.);
#4586=ADVANCED_FACE('',(#673),#496,.T.);
#4587=ADVANCED_FACE('',(#674),#4487,.F.);
#4588=ADVANCED_FACE('',(#675),#497,.F.);
#4589=ADVANCED_FACE('',(#676),#4488,.F.);
#4590=ADVANCED_FACE('',(#677),#498,.F.);
#4591=ADVANCED_FACE('',(#678),#4489,.F.);
#4592=ADVANCED_FACE('',(#679),#499,.F.);
#4593=ADVANCED_FACE('',(#680),#4490,.F.);
#4594=ADVANCED_FACE('',(#681),#500,.F.);
#4595=ADVANCED_FACE('',(#682),#4491,.F.);
#4596=ADVANCED_FACE('',(#683),#4492,.F.);
#4597=ADVANCED_FACE('',(#684),#4493,.F.);
#4598=ADVANCED_FACE('',(#685),#4494,.F.);
#4599=ADVANCED_FACE('',(#686),#4495,.F.);
#4600=ADVANCED_FACE('',(#687),#501,.T.);
#4601=ADVANCED_FACE('',(#688),#502,.T.);
#4602=ADVANCED_FACE('',(#689),#503,.F.);
#4603=ADVANCED_FACE('',(#690),#504,.F.);
#4604=ADVANCED_FACE('',(#691,#388),#505,.T.);
#4605=ADVANCED_FACE('',(#692,#389),#506,.T.);
#4606=ADVANCED_FACE('',(#693),#507,.T.);
#4607=ADVANCED_FACE('',(#694,#390,#391),#508,.T.);
#4608=ADVANCED_FACE('',(#695),#509,.T.);
#4609=ADVANCED_FACE('',(#696),#510,.T.);
#4610=ADVANCED_FACE('',(#697),#511,.T.);
#4611=ADVANCED_FACE('',(#698),#512,.F.);
#4612=ADVANCED_FACE('',(#699),#513,.F.);
#4613=ADVANCED_FACE('',(#700,#392),#514,.T.);
#4614=ADVANCED_FACE('',(#701,#393),#515,.T.);
#4615=ADVANCED_FACE('',(#702),#516,.T.);
#4616=ADVANCED_FACE('',(#703,#394,#395),#517,.T.);
#4617=ADVANCED_FACE('',(#704),#518,.T.);
#4618=ADVANCED_FACE('',(#705,#396),#4496,.F.);
#4619=ADVANCED_FACE('',(#706,#397,#398,#399),#4497,.T.);
#4620=ADVANCED_FACE('',(#707,#400,#401,#402,#403,#404),#519,.T.);
#4621=ADVANCED_FACE('',(#708,#405,#406,#407,#408,#409),#520,.F.);
#4869=CLOSED_SHELL('',(#4579,#4580,#4581,#4582,#4583,#4584,#4585,#4586,
#4587,#4588,#4589,#4590,#4591,#4592,#4593,#4594,#4595,#4596,#4597,#4598,
#4599,#4600,#4601,#4602,#4603,#4604,#4605,#4606,#4607,#4608,#4609,#4610,
#4611,#4612,#4613,#4614,#4615,#4616,#4617,#4618,#4619,#4620,#4621));
#5225=AXIS2_PLACEMENT_3D('',#7449,#5886,#5887);
#5226=AXIS2_PLACEMENT_3D('',#7450,#5888,#5889);
#5227=AXIS2_PLACEMENT_3D('',#7452,#5890,#5891);
#5228=AXIS2_PLACEMENT_3D('',#7455,#5893,#5894);
#5229=AXIS2_PLACEMENT_3D('',#7456,#5895,#5896);
#5230=AXIS2_PLACEMENT_3D('',#7457,#5897,#5898);
#5231=AXIS2_PLACEMENT_3D('',#7459,#5899,#5900);
#5232=AXIS2_PLACEMENT_3D('',#7462,#5902,#5903);
#5233=AXIS2_PLACEMENT_3D('',#7463,#5904,#5905);
#5234=AXIS2_PLACEMENT_3D('',#7464,#5906,#5907);
#5235=AXIS2_PLACEMENT_3D('',#7466,#5908,#5909);
#5236=AXIS2_PLACEMENT_3D('',#7469,#5911,#5912);
#5237=AXIS2_PLACEMENT_3D('',#7470,#5913,#5914);
#5238=AXIS2_PLACEMENT_3D('',#7471,#5915,#5916);
#5239=AXIS2_PLACEMENT_3D('',#7473,#5917,#5918);
#5240=AXIS2_PLACEMENT_3D('',#7476,#5920,#5921);
#5241=AXIS2_PLACEMENT_3D('',#7477,#5922,#5923);
#5242=AXIS2_PLACEMENT_3D('',#7478,#5924,#5925);
#5243=AXIS2_PLACEMENT_3D('',#7480,#5926,#5927);
#5244=AXIS2_PLACEMENT_3D('',#7483,#5929,#5930);
#5245=AXIS2_PLACEMENT_3D('',#7484,#5931,#5932);
#5246=AXIS2_PLACEMENT_3D('',#7485,#5933,#5934);
#5247=AXIS2_PLACEMENT_3D('',#7487,#5935,#5936);
#5248=AXIS2_PLACEMENT_3D('',#7490,#5938,#5939);
#5249=AXIS2_PLACEMENT_3D('',#7491,#5940,#5941);
#5250=AXIS2_PLACEMENT_3D('',#7492,#5942,#5943);
#5251=AXIS2_PLACEMENT_3D('',#7494,#5944,#5945);
#5252=AXIS2_PLACEMENT_3D('',#7497,#5947,#5948);
#5253=AXIS2_PLACEMENT_3D('',#7498,#5949,#5950);
#5254=AXIS2_PLACEMENT_3D('',#7499,#5951,#5952);
#5255=AXIS2_PLACEMENT_3D('',#7501,#5953,#5954);
#5256=AXIS2_PLACEMENT_3D('',#7504,#5956,#5957);
#5257=AXIS2_PLACEMENT_3D('',#7505,#5958,#5959);
#5258=AXIS2_PLACEMENT_3D('',#7506,#5960,#5961);
#5259=AXIS2_PLACEMENT_3D('',#7584,#5963,#5964);
#5260=AXIS2_PLACEMENT_3D('',#7586,#5965,#5966);
#5261=AXIS2_PLACEMENT_3D('',#7589,#5968,#5969);
#5262=AXIS2_PLACEMENT_3D('',#7590,#5970,#5971);
#5263=AXIS2_PLACEMENT_3D('',#7592,#5972,#5973);
#5264=AXIS2_PLACEMENT_3D('',#7595,#5975,#5976);
#5265=AXIS2_PLACEMENT_3D('',#7596,#5977,#5978);
#5266=AXIS2_PLACEMENT_3D('',#7598,#5979,#5980);
#5267=AXIS2_PLACEMENT_3D('',#7601,#5982,#5983);
#5268=AXIS2_PLACEMENT_3D('',#7602,#5984,#5985);
#5269=AXIS2_PLACEMENT_3D('',#7604,#5986,#5987);
#5270=AXIS2_PLACEMENT_3D('',#7607,#5989,#5990);
#5271=AXIS2_PLACEMENT_3D('',#7608,#5991,#5992);
#5272=AXIS2_PLACEMENT_3D('',#7611,#5993,#5994);
#5273=AXIS2_PLACEMENT_3D('',#7617,#5998,#5999);
#5274=AXIS2_PLACEMENT_3D('',#7619,#6000,#6001);
#5275=AXIS2_PLACEMENT_3D('',#7625,#6005,#6006);
#5276=AXIS2_PLACEMENT_3D('',#7628,#6007,#6008);
#5277=AXIS2_PLACEMENT_3D('',#7634,#6012,#6013);
#5278=AXIS2_PLACEMENT_3D('',#7636,#6014,#6015);
#5279=AXIS2_PLACEMENT_3D('',#7642,#6019,#6020);
#5280=AXIS2_PLACEMENT_3D('',#7645,#6023,#6024);
#5281=AXIS2_PLACEMENT_3D('',#7648,#6027,#6028);
#5282=AXIS2_PLACEMENT_3D('',#7650,#6030,#6031);
#5283=AXIS2_PLACEMENT_3D('',#7652,#6033,#6034);
#5284=AXIS2_PLACEMENT_3D('',#7653,#6035,#6036);
#5285=AXIS2_PLACEMENT_3D('',#7656,#6037,#6038);
#5286=AXIS2_PLACEMENT_3D('',#7662,#6042,#6043);
#5287=AXIS2_PLACEMENT_3D('',#7664,#6044,#6045);
#5288=AXIS2_PLACEMENT_3D('',#7670,#6049,#6050);
#5289=AXIS2_PLACEMENT_3D('',#7673,#6051,#6052);
#5290=AXIS2_PLACEMENT_3D('',#7679,#6056,#6057);
#5291=AXIS2_PLACEMENT_3D('',#7681,#6058,#6059);
#5292=AXIS2_PLACEMENT_3D('',#7687,#6063,#6064);
#5293=AXIS2_PLACEMENT_3D('',#7690,#6067,#6068);
#5294=AXIS2_PLACEMENT_3D('',#7693,#6071,#6072);
#5295=AXIS2_PLACEMENT_3D('',#7695,#6074,#6075);
#5296=AXIS2_PLACEMENT_3D('',#7697,#6077,#6078);
#5297=AXIS2_PLACEMENT_3D('',#7698,#6079,#6080);
#5298=AXIS2_PLACEMENT_3D('',#7700,#6081,#6082);
#5299=AXIS2_PLACEMENT_3D('',#7703,#6084,#6085);
#5300=AXIS2_PLACEMENT_3D('',#7704,#6086,#6087);
#5301=AXIS2_PLACEMENT_3D('',#7706,#6088,#6089);
#5302=AXIS2_PLACEMENT_3D('',#7709,#6091,#6092);
#5303=AXIS2_PLACEMENT_3D('',#7710,#6093,#6094);
#5304=AXIS2_PLACEMENT_3D('',#7711,#6095,#6096);
#5886=DIRECTION('axis',(0.,0.,1.));
#5887=DIRECTION('refdir',(1.,0.,0.));
#5888=DIRECTION('center_axis',(0.,1.,0.));
#5889=DIRECTION('ref_axis',(1.,0.,0.));
#5890=DIRECTION('center_axis',(0.,1.,0.));
#5891=DIRECTION('ref_axis',(1.,0.,0.));
#5892=DIRECTION('',(0.,1.,0.));
#5893=DIRECTION('center_axis',(0.,-1.,0.));
#5894=DIRECTION('ref_axis',(1.,0.,0.));
#5895=DIRECTION('center_axis',(0.,1.,0.));
#5896=DIRECTION('ref_axis',(1.,0.,0.));
#5897=DIRECTION('center_axis',(0.,1.,0.));
#5898=DIRECTION('ref_axis',(1.,0.,0.));
#5899=DIRECTION('center_axis',(0.,1.,0.));
#5900=DIRECTION('ref_axis',(1.,0.,0.));
#5901=DIRECTION('',(0.,1.,0.));
#5902=DIRECTION('center_axis',(0.,-1.,0.));
#5903=DIRECTION('ref_axis',(1.,0.,0.));
#5904=DIRECTION('center_axis',(0.,1.,0.));
#5905=DIRECTION('ref_axis',(1.,0.,0.));
#5906=DIRECTION('center_axis',(0.,1.,0.));
#5907=DIRECTION('ref_axis',(1.,0.,0.));
#5908=DIRECTION('center_axis',(0.,1.,0.));
#5909=DIRECTION('ref_axis',(1.,0.,0.));
#5910=DIRECTION('',(0.,1.,0.));
#5911=DIRECTION('center_axis',(0.,-1.,0.));
#5912=DIRECTION('ref_axis',(1.,0.,0.));
#5913=DIRECTION('center_axis',(0.,1.,0.));
#5914=DIRECTION('ref_axis',(1.,0.,0.));
#5915=DIRECTION('center_axis',(0.,1.,0.));
#5916=DIRECTION('ref_axis',(1.,0.,0.));
#5917=DIRECTION('center_axis',(0.,1.,0.));
#5918=DIRECTION('ref_axis',(1.,0.,0.));
#5919=DIRECTION('',(0.,1.,0.));
#5920=DIRECTION('center_axis',(0.,-1.,0.));
#5921=DIRECTION('ref_axis',(1.,0.,0.));
#5922=DIRECTION('center_axis',(0.,1.,0.));
#5923=DIRECTION('ref_axis',(1.,0.,0.));
#5924=DIRECTION('center_axis',(0.,1.,0.));
#5925=DIRECTION('ref_axis',(1.,0.,0.));
#5926=DIRECTION('center_axis',(0.,1.,0.));
#5927=DIRECTION('ref_axis',(1.,0.,0.));
#5928=DIRECTION('',(0.,1.,0.));
#5929=DIRECTION('center_axis',(0.,1.,0.));
#5930=DIRECTION('ref_axis',(1.,0.,0.));
#5931=DIRECTION('center_axis',(0.,1.,0.));
#5932=DIRECTION('ref_axis',(1.,0.,0.));
#5933=DIRECTION('center_axis',(0.,1.,0.));
#5934=DIRECTION('ref_axis',(1.,0.,0.));
#5935=DIRECTION('center_axis',(0.,1.,0.));
#5936=DIRECTION('ref_axis',(1.,0.,0.));
#5937=DIRECTION('',(0.,1.,0.));
#5938=DIRECTION('center_axis',(0.,1.,0.));
#5939=DIRECTION('ref_axis',(1.,0.,0.));
#5940=DIRECTION('center_axis',(0.,1.,0.));
#5941=DIRECTION('ref_axis',(1.,0.,0.));
#5942=DIRECTION('center_axis',(0.,1.,0.));
#5943=DIRECTION('ref_axis',(1.,0.,0.));
#5944=DIRECTION('center_axis',(0.,1.,0.));
#5945=DIRECTION('ref_axis',(1.,0.,0.));
#5946=DIRECTION('',(0.,1.,0.));
#5947=DIRECTION('center_axis',(0.,1.,0.));
#5948=DIRECTION('ref_axis',(1.,0.,0.));
#5949=DIRECTION('center_axis',(0.,1.,0.));
#5950=DIRECTION('ref_axis',(1.,0.,0.));
#5951=DIRECTION('center_axis',(0.,1.,0.));
#5952=DIRECTION('ref_axis',(1.,0.,0.));
#5953=DIRECTION('center_axis',(0.,1.,0.));
#5954=DIRECTION('ref_axis',(1.,0.,0.));
#5955=DIRECTION('',(0.,1.,0.));
#5956=DIRECTION('center_axis',(0.,1.,0.));
#5957=DIRECTION('ref_axis',(1.,0.,0.));
#5958=DIRECTION('center_axis',(0.,1.,0.));
#5959=DIRECTION('ref_axis',(1.,0.,0.));
#5960=DIRECTION('center_axis',(1.,0.,0.));
#5961=DIRECTION('ref_axis',(0.,0.,-1.));
#5962=DIRECTION('',(1.,0.,0.));
#5963=DIRECTION('center_axis',(0.,0.,1.));
#5964=DIRECTION('ref_axis',(1.,0.,0.));
#5965=DIRECTION('center_axis',(0.,0.,1.));
#5966=DIRECTION('ref_axis',(1.,0.,0.));
#5967=DIRECTION('',(0.,0.,1.));
#5968=DIRECTION('center_axis',(0.,0.,-1.));
#5969=DIRECTION('ref_axis',(1.,0.,0.));
#5970=DIRECTION('center_axis',(0.,0.,1.));
#5971=DIRECTION('ref_axis',(1.,0.,0.));
#5972=DIRECTION('center_axis',(0.,0.,1.));
#5973=DIRECTION('ref_axis',(1.,0.,0.));
#5974=DIRECTION('',(0.,0.,1.));
#5975=DIRECTION('center_axis',(0.,0.,-1.));
#5976=DIRECTION('ref_axis',(1.,0.,0.));
#5977=DIRECTION('center_axis',(0.,0.,1.));
#5978=DIRECTION('ref_axis',(1.,0.,0.));
#5979=DIRECTION('center_axis',(0.,0.,1.));
#5980=DIRECTION('ref_axis',(1.,0.,0.));
#5981=DIRECTION('',(0.,0.,1.));
#5982=DIRECTION('center_axis',(0.,0.,-1.));
#5983=DIRECTION('ref_axis',(1.,0.,0.));
#5984=DIRECTION('center_axis',(0.,0.,1.));
#5985=DIRECTION('ref_axis',(1.,0.,0.));
#5986=DIRECTION('center_axis',(0.,0.,1.));
#5987=DIRECTION('ref_axis',(1.,0.,0.));
#5988=DIRECTION('',(0.,0.,1.));
#5989=DIRECTION('center_axis',(0.,0.,-1.));
#5990=DIRECTION('ref_axis',(1.,0.,0.));
#5991=DIRECTION('center_axis',(0.,1.,0.));
#5992=DIRECTION('ref_axis',(0.,0.,1.));
#5993=DIRECTION('center_axis',(0.,1.,0.));
#5994=DIRECTION('ref_axis',(1.,0.,0.));
#5995=DIRECTION('',(1.,0.,0.));
#5996=DIRECTION('',(0.,0.,-1.));
#5997=DIRECTION('',(-1.,0.,0.));
#5998=DIRECTION('center_axis',(0.,1.,0.));
#5999=DIRECTION('ref_axis',(0.,0.,1.));
#6000=DIRECTION('center_axis',(0.,1.,0.));
#6001=DIRECTION('ref_axis',(1.,0.,0.));
#6002=DIRECTION('',(-1.,0.,0.));
#6003=DIRECTION('',(0.,0.,1.));
#6004=DIRECTION('',(1.,0.,0.));
#6005=DIRECTION('center_axis',(0.,1.,0.));
#6006=DIRECTION('ref_axis',(1.,0.,0.));
#6007=DIRECTION('center_axis',(0.,-1.,0.));
#6008=DIRECTION('ref_axis',(1.,0.,0.));
#6009=DIRECTION('',(1.,0.,0.));
#6010=DIRECTION('',(0.,0.,1.));
#6011=DIRECTION('',(-1.,0.,0.));
#6012=DIRECTION('center_axis',(0.,1.,0.));
#6013=DIRECTION('ref_axis',(1.,0.,0.));
#6014=DIRECTION('center_axis',(0.,-1.,0.));
#6015=DIRECTION('ref_axis',(1.,0.,0.));
#6016=DIRECTION('',(-1.,0.,0.));
#6017=DIRECTION('',(0.,0.,-1.));
#6018=DIRECTION('',(1.,0.,0.));
#6019=DIRECTION('center_axis',(0.,0.,1.));
#6020=DIRECTION('ref_axis',(1.,0.,0.));
#6021=DIRECTION('',(0.,1.,0.));
#6022=DIRECTION('',(0.,1.,0.));
#6023=DIRECTION('center_axis',(0.,0.,1.));
#6024=DIRECTION('ref_axis',(1.,0.,0.));
#6025=DIRECTION('',(0.,-1.,0.));
#6026=DIRECTION('',(0.,1.,0.));
#6027=DIRECTION('center_axis',(-1.,0.,0.));
#6028=DIRECTION('ref_axis',(0.,0.,1.));
#6029=DIRECTION('',(0.,1.,0.));
#6030=DIRECTION('center_axis',(0.,0.,-1.));
#6031=DIRECTION('ref_axis',(-1.,0.,0.));
#6032=DIRECTION('',(0.,1.,0.));
#6033=DIRECTION('center_axis',(1.,0.,0.));
#6034=DIRECTION('ref_axis',(0.,0.,-1.));
#6035=DIRECTION('center_axis',(0.,1.,0.));
#6036=DIRECTION('ref_axis',(0.,0.,1.));
#6037=DIRECTION('center_axis',(0.,1.,0.));
#6038=DIRECTION('ref_axis',(1.,0.,0.));
#6039=DIRECTION('',(1.,0.,0.));
#6040=DIRECTION('',(0.,0.,-1.));
#6041=DIRECTION('',(-1.,0.,0.));
#6042=DIRECTION('center_axis',(0.,1.,0.));
#6043=DIRECTION('ref_axis',(0.,0.,1.));
#6044=DIRECTION('center_axis',(0.,1.,0.));
#6045=DIRECTION('ref_axis',(1.,0.,0.));
#6046=DIRECTION('',(-1.,0.,0.));
#6047=DIRECTION('',(0.,0.,1.));
#6048=DIRECTION('',(1.,0.,0.));
#6049=DIRECTION('center_axis',(0.,1.,0.));
#6050=DIRECTION('ref_axis',(1.,0.,0.));
#6051=DIRECTION('center_axis',(0.,-1.,0.));
#6052=DIRECTION('ref_axis',(1.,0.,0.));
#6053=DIRECTION('',(1.,0.,0.));
#6054=DIRECTION('',(0.,0.,1.));
#6055=DIRECTION('',(-1.,0.,0.));
#6056=DIRECTION('center_axis',(0.,1.,0.));
#6057=DIRECTION('ref_axis',(1.,0.,0.));
#6058=DIRECTION('center_axis',(0.,-1.,0.));
#6059=DIRECTION('ref_axis',(1.,0.,0.));
#6060=DIRECTION('',(-1.,0.,0.));
#6061=DIRECTION('',(0.,0.,-1.));
#6062=DIRECTION('',(1.,0.,0.));
#6063=DIRECTION('center_axis',(0.,0.,1.));
#6064=DIRECTION('ref_axis',(1.,0.,0.));
#6065=DIRECTION('',(0.,1.,0.));
#6066=DIRECTION('',(0.,1.,0.));
#6067=DIRECTION('center_axis',(0.,0.,1.));
#6068=DIRECTION('ref_axis',(1.,0.,0.));
#6069=DIRECTION('',(0.,-1.,0.));
#6070=DIRECTION('',(0.,1.,0.));
#6071=DIRECTION('center_axis',(-1.,0.,0.));
#6072=DIRECTION('ref_axis',(0.,0.,1.));
#6073=DIRECTION('',(0.,1.,0.));
#6074=DIRECTION('center_axis',(0.,0.,-1.));
#6075=DIRECTION('ref_axis',(-1.,0.,0.));
#6076=DIRECTION('',(0.,1.,0.));
#6077=DIRECTION('center_axis',(1.,0.,0.));
#6078=DIRECTION('ref_axis',(0.,0.,-1.));
#6079=DIRECTION('center_axis',(0.,1.,0.));
#6080=DIRECTION('ref_axis',(1.,0.,0.));
#6081=DIRECTION('center_axis',(0.,-1.,0.));
#6082=DIRECTION('ref_axis',(1.,0.,0.));
#6083=DIRECTION('',(0.,-1.,0.));
#6084=DIRECTION('center_axis',(0.,-1.,0.));
#6085=DIRECTION('ref_axis',(1.,0.,0.));
#6086=DIRECTION('center_axis',(0.,1.,0.));
#6087=DIRECTION('ref_axis',(1.,0.,0.));
#6088=DIRECTION('center_axis',(0.,1.,0.));
#6089=DIRECTION('ref_axis',(1.,0.,0.));
#6090=DIRECTION('',(0.,-1.,0.));
#6091=DIRECTION('center_axis',(0.,1.,0.));
#6092=DIRECTION('ref_axis',(1.,0.,0.));
#6093=DIRECTION('center_axis',(0.,1.,0.));
#6094=DIRECTION('ref_axis',(1.,0.,0.));
#6095=DIRECTION('center_axis',(0.,1.,0.));
#6096=DIRECTION('ref_axis',(1.,0.,0.));
#7449=CARTESIAN_POINT('',(0.,0.,0.));
#7450=CARTESIAN_POINT('Origin',(-2.8,4.4,4.5));
#7451=CARTESIAN_POINT('',(-2.965,4.4,4.5));
#7452=CARTESIAN_POINT('Origin',(-2.8,4.4,4.5));
#7453=CARTESIAN_POINT('',(-2.965,6.,4.5));
#7454=CARTESIAN_POINT('',(-2.965,4.4,4.5));
#7455=CARTESIAN_POINT('Origin',(-2.8,6.,4.5));
#7456=CARTESIAN_POINT('Origin',(-2.8,4.4,4.5));
#7457=CARTESIAN_POINT('Origin',(1.71450551880629E-16,4.4,7.3));
#7458=CARTESIAN_POINT('',(-0.165,4.4,7.3));
#7459=CARTESIAN_POINT('Origin',(1.71450551880629E-16,4.4,7.3));
#7460=CARTESIAN_POINT('',(-0.165,6.,7.3));
#7461=CARTESIAN_POINT('',(-0.165,4.4,7.3));
#7462=CARTESIAN_POINT('Origin',(1.71450551880629E-16,6.,7.3));
#7463=CARTESIAN_POINT('Origin',(1.66533453693773E-16,4.4,7.3));
#7464=CARTESIAN_POINT('Origin',(2.8,4.4,4.5));
#7465=CARTESIAN_POINT('',(2.635,4.4,4.5));
#7466=CARTESIAN_POINT('Origin',(2.8,4.4,4.5));
#7467=CARTESIAN_POINT('',(2.635,6.,4.5));
#7468=CARTESIAN_POINT('',(2.635,4.4,4.5));
#7469=CARTESIAN_POINT('Origin',(2.8,6.,4.5));
#7470=CARTESIAN_POINT('Origin',(2.8,4.4,4.5));
#7471=CARTESIAN_POINT('Origin',(-5.14351655641888E-16,4.4,1.7));
#7472=CARTESIAN_POINT('',(-0.165000000000001,4.4,1.7));
#7473=CARTESIAN_POINT('Origin',(-5.14351655641888E-16,4.4,1.7));
#7474=CARTESIAN_POINT('',(-0.165000000000001,6.,1.7));
#7475=CARTESIAN_POINT('',(-0.165000000000001,4.4,1.7));
#7476=CARTESIAN_POINT('Origin',(-5.14351655641888E-16,6.,1.7));
#7477=CARTESIAN_POINT('Origin',(-5.27355936696949E-16,4.4,1.7));
#7478=CARTESIAN_POINT('Origin',(-2.8,-0.1,4.5));
#7479=CARTESIAN_POINT('',(-2.965,0.,4.5));
#7480=CARTESIAN_POINT('Origin',(-2.8,0.,4.5));
#7481=CARTESIAN_POINT('',(-2.965,1.6,4.5));
#7482=CARTESIAN_POINT('',(-2.965,-0.1,4.5));
#7483=CARTESIAN_POINT('Origin',(-2.8,1.6,4.5));
#7484=CARTESIAN_POINT('Origin',(-2.8,1.6,4.5));
#7485=CARTESIAN_POINT('Origin',(1.71450551880629E-16,-0.1,7.3));
#7486=CARTESIAN_POINT('',(-0.165,0.,7.3));
#7487=CARTESIAN_POINT('Origin',(1.71450551880629E-16,0.,7.3));
#7488=CARTESIAN_POINT('',(-0.165,1.6,7.3));
#7489=CARTESIAN_POINT('',(-0.165,-0.1,7.3));
#7490=CARTESIAN_POINT('Origin',(1.71450551880629E-16,1.6,7.3));
#7491=CARTESIAN_POINT('Origin',(1.66533453693773E-16,1.6,7.3));
#7492=CARTESIAN_POINT('Origin',(2.8,-0.1,4.5));
#7493=CARTESIAN_POINT('',(2.635,0.,4.5));
#7494=CARTESIAN_POINT('Origin',(2.8,0.,4.5));
#7495=CARTESIAN_POINT('',(2.635,1.6,4.5));
#7496=CARTESIAN_POINT('',(2.635,-0.1,4.5));
#7497=CARTESIAN_POINT('Origin',(2.8,1.6,4.5));
#7498=CARTESIAN_POINT('Origin',(2.8,1.6,4.5));
#7499=CARTESIAN_POINT('Origin',(-5.14351655641888E-16,-0.1,1.7));
#7500=CARTESIAN_POINT('',(-0.165000000000001,0.,1.7));
#7501=CARTESIAN_POINT('Origin',(-5.14351655641888E-16,0.,1.7));
#7502=CARTESIAN_POINT('',(-0.165000000000001,1.6,1.7));
#7503=CARTESIAN_POINT('',(-0.165000000000001,-0.1,1.7));
#7504=CARTESIAN_POINT('Origin',(-5.14351655641888E-16,1.6,1.7));
#7505=CARTESIAN_POINT('Origin',(-5.27355936696949E-16,1.6,1.7));
#7506=CARTESIAN_POINT('Origin',(2.1,3.,4.5));
#7507=CARTESIAN_POINT('',(2.24794906525926,3.,3.815));
#7508=CARTESIAN_POINT('',(2.24794906525926,3.,5.185));
#7509=CARTESIAN_POINT('Ctrl Pts',(2.24794906525926,3.,3.815));
#7510=CARTESIAN_POINT('Ctrl Pts',(2.24794906525926,3.08656638593426,3.815));
#7511=CARTESIAN_POINT('Ctrl Pts',(2.25347242618579,3.1785329272349,3.83240366255852));
#7512=CARTESIAN_POINT('Ctrl Pts',(2.273052742601,3.34713817113353,3.90246002212197));
#7513=CARTESIAN_POINT('Ctrl Pts',(2.28678795375575,3.42382433348001,3.95508804325444));
#7514=CARTESIAN_POINT('Ctrl Pts',(2.31229010718961,3.54489596201988,4.07615967179431));
#7515=CARTESIAN_POINT('Ctrl Pts',(2.32576600179013,3.59753638520302,4.15285236357336));
#7516=CARTESIAN_POINT('Ctrl Pts',(2.34474519428597,3.66760188102413,4.32148123334598));
#7517=CARTESIAN_POINT('Ctrl Pts',(2.35,3.685,4.4134564835475));
#7518=CARTESIAN_POINT('Ctrl Pts',(2.35,3.685,4.5865435164525));
#7519=CARTESIAN_POINT('Ctrl Pts',(2.34474519428597,3.66760188102413,4.67851876665402));
#7520=CARTESIAN_POINT('Ctrl Pts',(2.32576600179013,3.59753638520302,4.84714763642664));
#7521=CARTESIAN_POINT('Ctrl Pts',(2.31229010718961,3.54489596201988,4.92384032820569));
#7522=CARTESIAN_POINT('Ctrl Pts',(2.28678795375575,3.42382433348001,5.04491195674555));
#7523=CARTESIAN_POINT('Ctrl Pts',(2.273052742601,3.34713817113353,5.09753997787803));
#7524=CARTESIAN_POINT('Ctrl Pts',(2.25347242618579,3.1785329272349,5.16759633744148));
#7525=CARTESIAN_POINT('Ctrl Pts',(2.24794906525926,3.08656638593426,5.185));
#7526=CARTESIAN_POINT('Ctrl Pts',(2.24794906525926,3.,5.185));
#7527=CARTESIAN_POINT('Ctrl Pts',(2.24794906525926,3.,5.185));
#7528=CARTESIAN_POINT('Ctrl Pts',(2.24794906525926,2.91343361406574,5.185));
#7529=CARTESIAN_POINT('Ctrl Pts',(2.25347242618579,2.8214670727651,5.16759633744148));
#7530=CARTESIAN_POINT('Ctrl Pts',(2.273052742601,2.65286182886647,5.09753997787803));
#7531=CARTESIAN_POINT('Ctrl Pts',(2.28678795375575,2.57617566651999,5.04491195674556));
#7532=CARTESIAN_POINT('Ctrl Pts',(2.31229010718961,2.45510403798012,4.92384032820569));
#7533=CARTESIAN_POINT('Ctrl Pts',(2.32576600179013,2.40246361479698,4.84714763642664));
#7534=CARTESIAN_POINT('Ctrl Pts',(2.34474519428597,2.33239811897587,4.67851876665402));
#7535=CARTESIAN_POINT('Ctrl Pts',(2.35,2.315,4.5865435164525));
#7536=CARTESIAN_POINT('Ctrl Pts',(2.35,2.315,4.4134564835475));
#7537=CARTESIAN_POINT('Ctrl Pts',(2.34474519428597,2.33239811897587,4.32148123334598));
#7538=CARTESIAN_POINT('Ctrl Pts',(2.32576600179013,2.40246361479698,4.15285236357336));
#7539=CARTESIAN_POINT('Ctrl Pts',(2.31229010718961,2.45510403798012,4.07615967179431));
#7540=CARTESIAN_POINT('Ctrl Pts',(2.28678795375575,2.57617566651999,3.95508804325444));
#7541=CARTESIAN_POINT('Ctrl Pts',(2.273052742601,2.65286182886647,3.90246002212197));
#7542=CARTESIAN_POINT('Ctrl Pts',(2.25347242618579,2.8214670727651,3.83240366255852));
#7543=CARTESIAN_POINT('Ctrl Pts',(2.24794906525926,2.91343361406574,3.815));
#7544=CARTESIAN_POINT('Ctrl Pts',(2.24794906525926,3.,3.815));
#7545=CARTESIAN_POINT('',(3.43231335982017,3.,5.185));
#7546=CARTESIAN_POINT('',(2.1,3.,5.185));
#7547=CARTESIAN_POINT('',(3.43231335982017,3.,3.815));
#7548=CARTESIAN_POINT('Ctrl Pts',(3.43231335982017,3.,3.815));
#7549=CARTESIAN_POINT('Ctrl Pts',(3.43231335982017,2.91374778588775,3.815));
#7550=CARTESIAN_POINT('Ctrl Pts',(3.43590159793026,2.82190332857989,3.83228322178306));
#7551=CARTESIAN_POINT('Ctrl Pts',(3.44876354740763,2.65320224067205,3.90225803271408));
#7552=CARTESIAN_POINT('Ctrl Pts',(3.45784079740304,2.57632582235222,3.95493788742221));
#7553=CARTESIAN_POINT('Ctrl Pts',(3.47480256335419,2.45494100103992,4.07632270873451));
#7554=CARTESIAN_POINT('Ctrl Pts',(3.48380333962794,2.40225870697367,4.15320045129105));
#7555=CARTESIAN_POINT('Ctrl Pts',(3.49648941236884,2.33228212593366,4.3219061343655));
#7556=CARTESIAN_POINT('Ctrl Pts',(3.5,2.315,4.41375221065075));
#7557=CARTESIAN_POINT('Ctrl Pts',(3.5,2.315,4.58624778934925));
#7558=CARTESIAN_POINT('Ctrl Pts',(3.49648941236884,2.33228212593366,4.6780938656345));
#7559=CARTESIAN_POINT('Ctrl Pts',(3.48380333962794,2.40225870697367,4.84679954870895));
#7560=CARTESIAN_POINT('Ctrl Pts',(3.47480256335419,2.45494100103992,4.92367729126549));
#7561=CARTESIAN_POINT('Ctrl Pts',(3.45784079740304,2.57632582235222,5.04506211257779));
#7562=CARTESIAN_POINT('Ctrl Pts',(3.44876354740763,2.65320224067205,5.09774196728592));
#7563=CARTESIAN_POINT('Ctrl Pts',(3.43590159793026,2.82190332857989,5.16771677821694));
#7564=CARTESIAN_POINT('Ctrl Pts',(3.43231335982017,2.91374778588775,5.185));
#7565=CARTESIAN_POINT('Ctrl Pts',(3.43231335982017,3.,5.185));
#7566=CARTESIAN_POINT('Ctrl Pts',(3.43231335982017,3.,5.185));
#7567=CARTESIAN_POINT('Ctrl Pts',(3.43231335982017,3.08625221411225,5.185));
#7568=CARTESIAN_POINT('Ctrl Pts',(3.43590159793026,3.17809667142011,5.16771677821694));
#7569=CARTESIAN_POINT('Ctrl Pts',(3.44876354740763,3.34679775932795,5.09774196728592));
#7570=CARTESIAN_POINT('Ctrl Pts',(3.45784079740304,3.42367417764778,5.04506211257779));
#7571=CARTESIAN_POINT('Ctrl Pts',(3.47480256335419,3.54505899896008,4.92367729126549));
#7572=CARTESIAN_POINT('Ctrl Pts',(3.48380333962794,3.59774129302633,4.84679954870895));
#7573=CARTESIAN_POINT('Ctrl Pts',(3.49648941236884,3.66771787406634,4.6780938656345));
#7574=CARTESIAN_POINT('Ctrl Pts',(3.5,3.685,4.58624778934925));
#7575=CARTESIAN_POINT('Ctrl Pts',(3.5,3.685,4.41375221065075));
#7576=CARTESIAN_POINT('Ctrl Pts',(3.49648941236884,3.66771787406634,4.3219061343655));
#7577=CARTESIAN_POINT('Ctrl Pts',(3.48380333962794,3.59774129302633,4.15320045129105));
#7578=CARTESIAN_POINT('Ctrl Pts',(3.47480256335419,3.54505899896008,4.07632270873451));
#7579=CARTESIAN_POINT('Ctrl Pts',(3.45784079740304,3.42367417764778,3.95493788742221));
#7580=CARTESIAN_POINT('Ctrl Pts',(3.44876354740763,3.34679775932795,3.90225803271408));
#7581=CARTESIAN_POINT('Ctrl Pts',(3.43590159793026,3.17809667142011,3.83228322178306));
#7582=CARTESIAN_POINT('Ctrl Pts',(3.43231335982017,3.08625221411225,3.815));
#7583=CARTESIAN_POINT('Ctrl Pts',(3.43231335982017,3.,3.815));
#7584=CARTESIAN_POINT('Origin',(3.8,1.,0.9));
#7585=CARTESIAN_POINT('',(3.47,1.,1.));
#7586=CARTESIAN_POINT('Origin',(3.8,1.,1.));
#7587=CARTESIAN_POINT('',(3.47,1.,2.5));
#7588=CARTESIAN_POINT('',(3.47,1.,0.9));
#7589=CARTESIAN_POINT('Origin',(3.8,1.,2.5));
#7590=CARTESIAN_POINT('Origin',(-3.8,5.,0.9));
#7591=CARTESIAN_POINT('',(-4.13,5.,1.));
#7592=CARTESIAN_POINT('Origin',(-3.8,5.,1.));
#7593=CARTESIAN_POINT('',(-4.13,5.,2.5));
#7594=CARTESIAN_POINT('',(-4.13,5.,0.9));
#7595=CARTESIAN_POINT('Origin',(-3.8,5.,2.5));
#7596=CARTESIAN_POINT('Origin',(-3.8,1.,0.9));
#7597=CARTESIAN_POINT('',(-4.13,1.,1.));
#7598=CARTESIAN_POINT('Origin',(-3.8,1.,1.));
#7599=CARTESIAN_POINT('',(-4.13,1.,2.5));
#7600=CARTESIAN_POINT('',(-4.13,1.,0.9));
#7601=CARTESIAN_POINT('Origin',(-3.8,1.,2.5));
#7602=CARTESIAN_POINT('Origin',(3.8,5.,0.9));
#7603=CARTESIAN_POINT('',(3.47,5.,1.));
#7604=CARTESIAN_POINT('Origin',(3.8,5.,1.));
#7605=CARTESIAN_POINT('',(3.47,5.,2.5));
#7606=CARTESIAN_POINT('',(3.47,5.,0.9));
#7607=CARTESIAN_POINT('Origin',(3.8,5.,2.5));
#7608=CARTESIAN_POINT('Origin',(0.,5.5,1.75));
#7609=CARTESIAN_POINT('',(2.87228132326901,5.5,2.5));
#7610=CARTESIAN_POINT('',(0.,5.5,1.));
#7611=CARTESIAN_POINT('Origin',(0.,5.5,4.5));
#7612=CARTESIAN_POINT('',(4.5,5.5,2.5));
#7613=CARTESIAN_POINT('',(4.5,5.5,2.5));
#7614=CARTESIAN_POINT('',(4.5,5.5,1.));
#7615=CARTESIAN_POINT('',(4.5,5.5,1.));
#7616=CARTESIAN_POINT('',(-4.5,5.5,1.));
#7617=CARTESIAN_POINT('Origin',(0.,5.5,1.75));
#7618=CARTESIAN_POINT('',(-2.87228132326901,5.5,2.5));
#7619=CARTESIAN_POINT('Origin',(0.,5.5,4.5));
#7620=CARTESIAN_POINT('',(-4.5,5.5,1.));
#7621=CARTESIAN_POINT('',(-4.5,5.5,1.));
#7622=CARTESIAN_POINT('',(-4.5,5.5,2.5));
#7623=CARTESIAN_POINT('',(-4.5,5.5,2.5));
#7624=CARTESIAN_POINT('',(4.5,5.5,2.5));
#7625=CARTESIAN_POINT('Origin',(0.,4.5,1.75));
#7626=CARTESIAN_POINT('',(0.,4.5,1.));
#7627=CARTESIAN_POINT('',(2.87228132326901,4.5,2.5));
#7628=CARTESIAN_POINT('Origin',(0.,4.5,4.5));
#7629=CARTESIAN_POINT('',(4.5,4.5,1.));
#7630=CARTESIAN_POINT('',(-4.5,4.5,1.));
#7631=CARTESIAN_POINT('',(4.5,4.5,2.5));
#7632=CARTESIAN_POINT('',(4.5,4.5,1.));
#7633=CARTESIAN_POINT('',(4.5,4.5,2.5));
#7634=CARTESIAN_POINT('Origin',(0.,4.5,1.75));
#7635=CARTESIAN_POINT('',(-2.87228132326901,4.5,2.5));
#7636=CARTESIAN_POINT('Origin',(0.,4.5,4.5));
#7637=CARTESIAN_POINT('',(-4.5,4.5,2.5));
#7638=CARTESIAN_POINT('',(4.5,4.5,2.5));
#7639=CARTESIAN_POINT('',(-4.5,4.5,1.));
#7640=CARTESIAN_POINT('',(-4.5,4.5,2.5));
#7641=CARTESIAN_POINT('',(-4.5,4.5,1.));
#7642=CARTESIAN_POINT('Origin',(-4.5,4.5,2.5));
#7643=CARTESIAN_POINT('',(2.87228132326901,0.,2.5));
#7644=CARTESIAN_POINT('',(4.5,4.5,2.5));
#7645=CARTESIAN_POINT('Origin',(-4.5,4.5,2.5));
#7646=CARTESIAN_POINT('',(-2.87228132326901,0.,2.5));
#7647=CARTESIAN_POINT('',(-4.5,4.5,2.5));
#7648=CARTESIAN_POINT('Origin',(-4.5,4.5,1.));
#7649=CARTESIAN_POINT('',(-4.5,4.5,1.));
#7650=CARTESIAN_POINT('Origin',(4.5,4.5,1.));
#7651=CARTESIAN_POINT('',(4.5,4.5,1.));
#7652=CARTESIAN_POINT('Origin',(4.5,4.5,2.5));
#7653=CARTESIAN_POINT('Origin',(0.,1.5,1.75));
#7654=CARTESIAN_POINT('',(2.87228132326901,1.5,2.5));
#7655=CARTESIAN_POINT('',(0.,1.5,1.));
#7656=CARTESIAN_POINT('Origin',(0.,1.5,4.5));
#7657=CARTESIAN_POINT('',(4.5,1.5,2.5));
#7658=CARTESIAN_POINT('',(4.5,1.5,2.5));
#7659=CARTESIAN_POINT('',(4.5,1.5,1.));
#7660=CARTESIAN_POINT('',(4.5,1.5,1.));
#7661=CARTESIAN_POINT('',(-4.5,1.5,1.));
#7662=CARTESIAN_POINT('Origin',(0.,1.5,1.75));
#7663=CARTESIAN_POINT('',(-2.87228132326901,1.5,2.5));
#7664=CARTESIAN_POINT('Origin',(0.,1.5,4.5));
#7665=CARTESIAN_POINT('',(-4.5,1.5,1.));
#7666=CARTESIAN_POINT('',(-4.5,1.5,1.));
#7667=CARTESIAN_POINT('',(-4.5,1.5,2.5));
#7668=CARTESIAN_POINT('',(-4.5,1.5,2.5));
#7669=CARTESIAN_POINT('',(4.5,1.5,2.5));
#7670=CARTESIAN_POINT('Origin',(0.,0.5,1.75));
#7671=CARTESIAN_POINT('',(0.,0.5,1.));
#7672=CARTESIAN_POINT('',(2.87228132326901,0.5,2.5));
#7673=CARTESIAN_POINT('Origin',(0.,0.5,4.5));
#7674=CARTESIAN_POINT('',(4.5,0.5,1.));
#7675=CARTESIAN_POINT('',(-4.5,0.5,1.));
#7676=CARTESIAN_POINT('',(4.5,0.5,2.5));
#7677=CARTESIAN_POINT('',(4.5,0.5,1.));
#7678=CARTESIAN_POINT('',(4.5,0.5,2.5));
#7679=CARTESIAN_POINT('Origin',(0.,0.5,1.75));
#7680=CARTESIAN_POINT('',(-2.87228132326901,0.5,2.5));
#7681=CARTESIAN_POINT('Origin',(0.,0.5,4.5));
#7682=CARTESIAN_POINT('',(-4.5,0.5,2.5));
#7683=CARTESIAN_POINT('',(4.5,0.5,2.5));
#7684=CARTESIAN_POINT('',(-4.5,0.5,1.));
#7685=CARTESIAN_POINT('',(-4.5,0.5,2.5));
#7686=CARTESIAN_POINT('',(-4.5,0.5,1.));
#7687=CARTESIAN_POINT('Origin',(-4.5,0.5,2.5));
#7688=CARTESIAN_POINT('',(2.87228132326901,0.,2.5));
#7689=CARTESIAN_POINT('',(4.5,0.5,2.5));
#7690=CARTESIAN_POINT('Origin',(-4.5,0.5,2.5));
#7691=CARTESIAN_POINT('',(-2.87228132326901,0.,2.5));
#7692=CARTESIAN_POINT('',(-4.5,0.5,2.5));
#7693=CARTESIAN_POINT('Origin',(-4.5,0.5,1.));
#7694=CARTESIAN_POINT('',(-4.5,0.5,1.));
#7695=CARTESIAN_POINT('Origin',(4.5,0.5,1.));
#7696=CARTESIAN_POINT('',(4.5,0.5,1.));
#7697=CARTESIAN_POINT('Origin',(4.5,0.5,2.5));
#7698=CARTESIAN_POINT('Origin',(0.,0.,4.5));
#7699=CARTESIAN_POINT('',(-2.35,6.,4.5));
#7700=CARTESIAN_POINT('Origin',(0.,6.,4.5));
#7701=CARTESIAN_POINT('',(-2.35,0.,4.5));
#7702=CARTESIAN_POINT('',(-2.35,0.,4.5));
#7703=CARTESIAN_POINT('Origin',(0.,0.,4.5));
#7704=CARTESIAN_POINT('Origin',(0.,0.,4.5));
#7705=CARTESIAN_POINT('',(-3.5,6.,4.5));
#7706=CARTESIAN_POINT('Origin',(0.,6.,4.5));
#7707=CARTESIAN_POINT('',(-3.5,0.,4.5));
#7708=CARTESIAN_POINT('',(-3.5,0.,4.5));
#7709=CARTESIAN_POINT('Origin',(0.,0.,4.5));
#7710=CARTESIAN_POINT('Origin',(0.,6.,4.5));
#7711=CARTESIAN_POINT('Origin',(0.,0.,4.5));
#9388=UNCERTAINTY_MEASURE_WITH_UNIT(LENGTH_MEASURE(0.001),#9449,
'DISTANCE_ACCURACY_VALUE',
'Maximum model space distance between geometric entities at asserted c
onnectivities');
#9416=UNCERTAINTY_MEASURE_WITH_UNIT(LENGTH_MEASURE(0.001),#9449,
'DISTANCE_ACCURACY_VALUE',
'Maximum model space distance between geometric entities at asserted c
onnectivities');
#9420=(
GEOMETRIC_REPRESENTATION_CONTEXT(3)
GLOBAL_UNCERTAINTY_ASSIGNED_CONTEXT((#9388))
GLOBAL_UNIT_ASSIGNED_CONTEXT((#9449,#9451,#9452))
REPRESENTATION_CONTEXT('','3D')
);
#9448=(
GEOMETRIC_REPRESENTATION_CONTEXT(3)
GLOBAL_UNCERTAINTY_ASSIGNED_CONTEXT((#9416))
GLOBAL_UNIT_ASSIGNED_CONTEXT((#9449,#9451,#9452))
REPRESENTATION_CONTEXT('','3D')
);
#9449=(
LENGTH_UNIT()
NAMED_UNIT(*)
SI_UNIT(.CENTI.,.METRE.)
);
#9451=(
NAMED_UNIT(*)
PLANE_ANGLE_UNIT()
SI_UNIT($,.RADIAN.)
);
#9452=(
NAMED_UNIT(*)
SI_UNIT($,.STERADIAN.)
SOLID_ANGLE_UNIT()
);
#9456=SHAPE_DEFINITION_REPRESENTATION(#9487,#9560);
#9487=PRODUCT_DEFINITION_SHAPE('',$,#9592);
#9560=SHAPE_REPRESENTATION('',(#5225),#9420);
#9588=PRODUCT_DEFINITION_CONTEXT('part definition',#9683,'design');
#9592=PRODUCT_DEFINITION('Housing','Housing',#9623,#9588);
#9623=PRODUCT_DEFINITION_FORMATION('',$,#9688);
#9683=APPLICATION_CONTEXT(
'Core Data for Automotive Mechanical Design Process');
#9684=PRODUCT_CONTEXT('part definition',#9683,'mechanical');
#9688=PRODUCT('Housing','Housing','Housing',(#9684));
#9751=COLOUR_RGB('Dark Blue',0.08,0.2,0.34);
#9752=FILL_AREA_STYLE_COLOUR('',#9751);
#9753=FILL_AREA_STYLE('',(#9752));
#9754=SURFACE_STYLE_FILL_AREA(#9753);
#9755=SURFACE_SIDE_STYLE('',(#9754));
#9756=SURFACE_STYLE_USAGE(.BOTH.,#9755);
#9757=PRESENTATION_STYLE_ASSIGNMENT((#9756));
ENDSEC;
END-ISO-10303-21;
